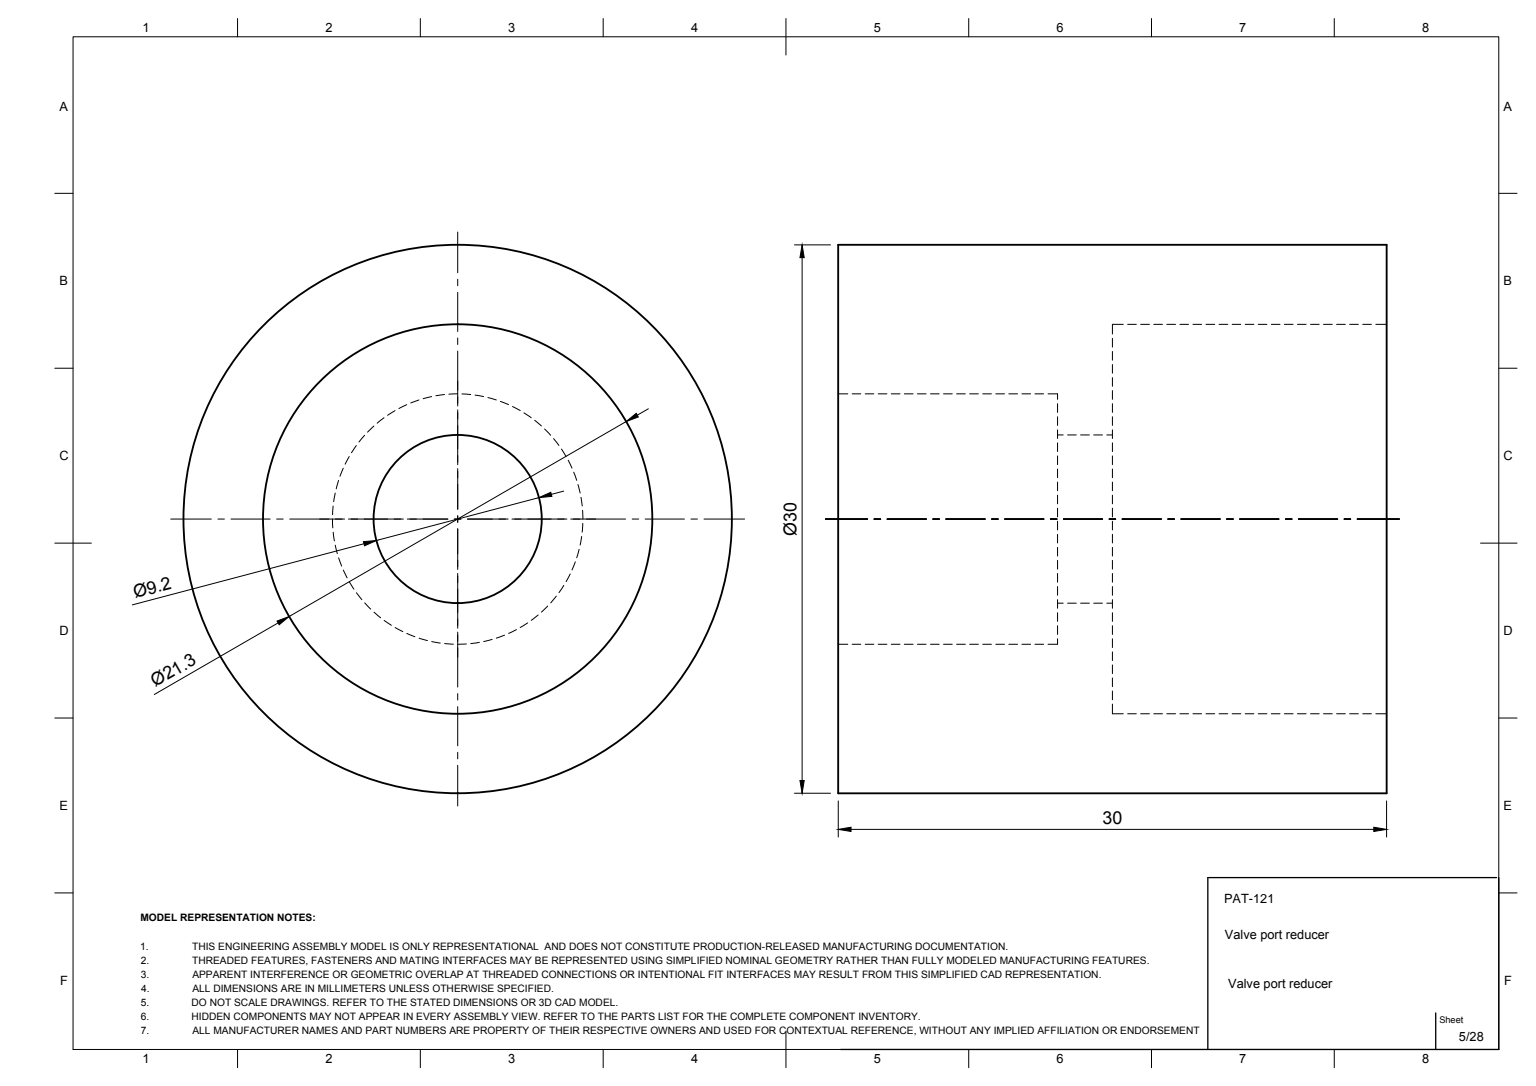
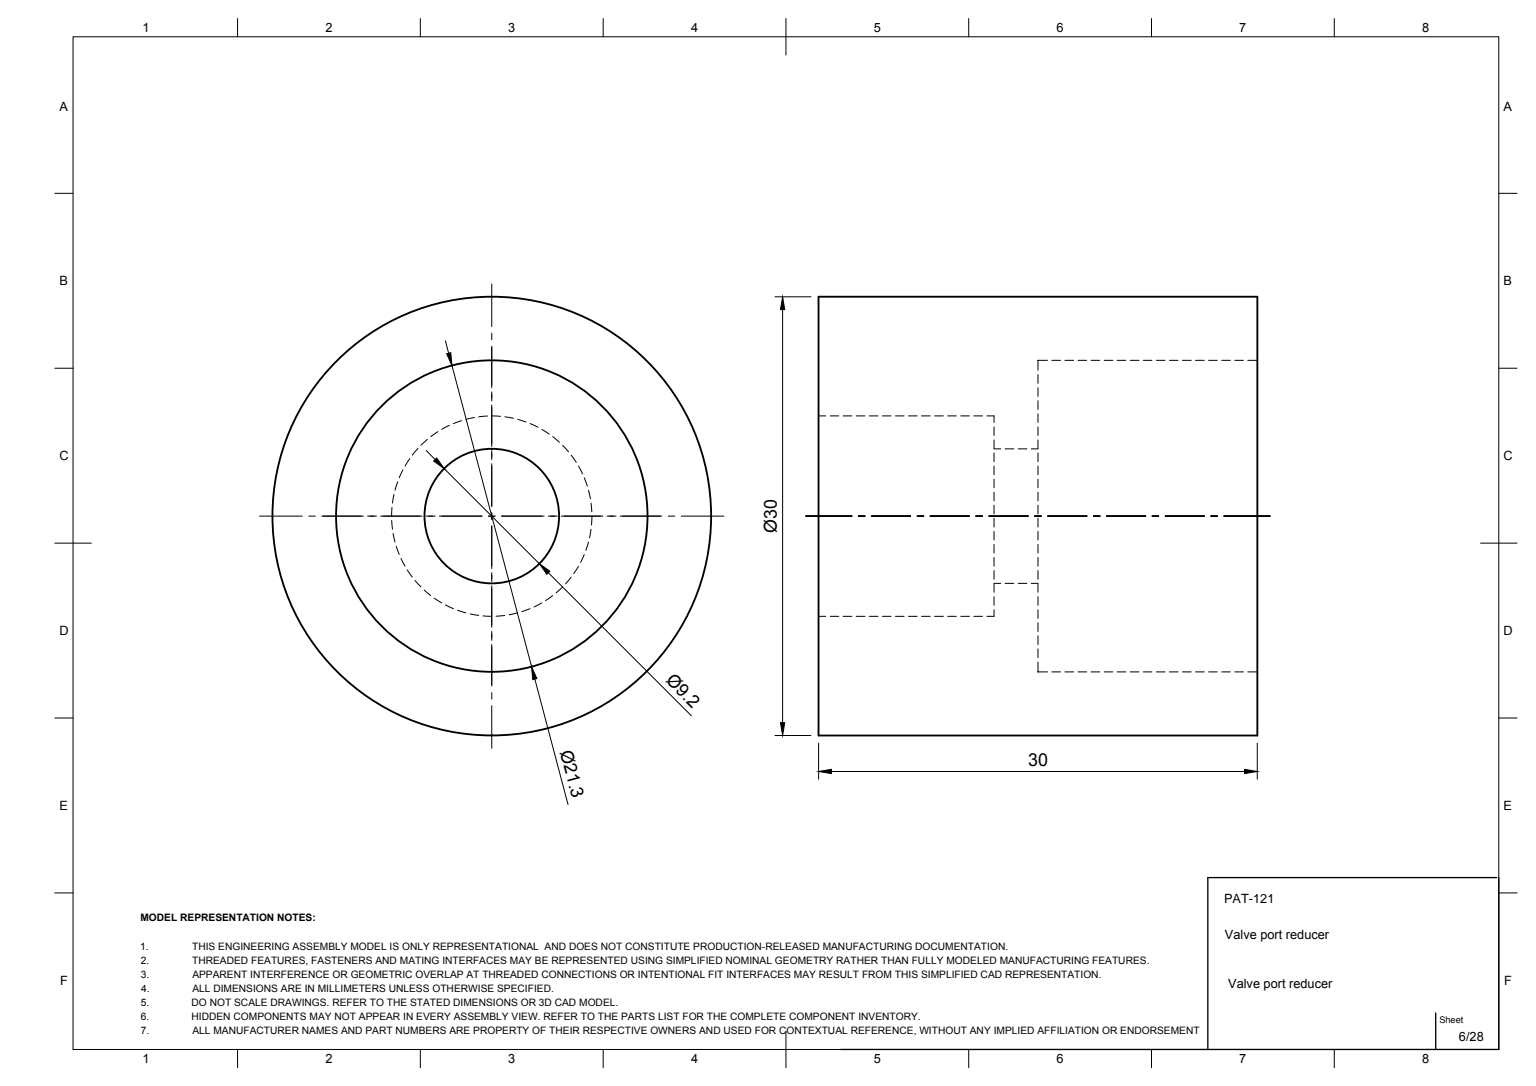
ISO-10303-21;
HEADER;
/* Generated by software containing ST-Developer
 * from STEP Tools, Inc. (www.steptools.com) 
 */

FILE_DESCRIPTION(
/* description */ ('Wall-mounted air drop station'),
/* implementation_level */ '2;1');

FILE_NAME(
/* name */ 'Valve port reducer.step',
/* time_stamp */ '2026-10-28T22:16:19-07:00',
/* author */ (''),
/* organization */ (''),
/* preprocessor_version */ 'ST-DEVELOPER v20.2',
/* originating_system */ 'Autodesk Translation Framework v15.17.0.0',
/* authorisation */ '');

FILE_SCHEMA (('AUTOMOTIVE_DESIGN { 1 0 10303 214 3 1 1 }'));
ENDSEC;

DATA;
#10=MECHANICAL_DESIGN_GEOMETRIC_PRESENTATION_REPRESENTATION('',(#344),#10517);
#286=SHAPE_REPRESENTATION_RELATIONSHIP('SRR','None',#10643,#315);
#315=ADVANCED_BREP_SHAPE_REPRESENTATION('',(#373),#10487);
#344=STYLED_ITEM('',(#10860),#373);
#373=MANIFOLD_SOLID_BREP('Body1',#5883);
#399=FACE_BOUND('',#1112,.T.);
#400=FACE_BOUND('',#1115,.T.);
#401=FACE_BOUND('',#1119,.T.);
#402=FACE_BOUND('',#1121,.T.);
#526=PLANE('',#6241);
#527=PLANE('',#6246);
#528=PLANE('',#6252);
#529=PLANE('',#6253);
#755=FACE_OUTER_BOUND('',#1110,.T.);
#756=FACE_OUTER_BOUND('',#1111,.T.);
#757=FACE_OUTER_BOUND('',#1113,.T.);
#758=FACE_OUTER_BOUND('',#1114,.T.);
#759=FACE_OUTER_BOUND('',#1116,.T.);
#760=FACE_OUTER_BOUND('',#1117,.T.);
#761=FACE_OUTER_BOUND('',#1118,.T.);
#762=FACE_OUTER_BOUND('',#1120,.T.);
#1110=EDGE_LOOP('',(#3973,#3974,#3975,#3976));
#1111=EDGE_LOOP('',(#3977));
#1112=EDGE_LOOP('',(#3978));
#1113=EDGE_LOOP('',(#3979,#3980,#3981,#3982));
#1114=EDGE_LOOP('',(#3983));
#1115=EDGE_LOOP('',(#3984));
#1116=EDGE_LOOP('',(#3985,#3986,#3987,#3988));
#1117=EDGE_LOOP('',(#3989,#3990,#3991,#3992));
#1118=EDGE_LOOP('',(#3993));
#1119=EDGE_LOOP('',(#3994));
#1120=EDGE_LOOP('',(#3995));
#1121=EDGE_LOOP('',(#3996));
#1592=LINE('',#8773,#2056);
#1593=LINE('',#8782,#2057);
#1594=LINE('',#8788,#2058);
#1595=LINE('',#8793,#2059);
#2056=VECTOR('',#6934,0.685);
#2057=VECTOR('',#6945,1.065);
#2058=VECTOR('',#6954,0.46);
#2059=VECTOR('',#6959,1.5);
#2520=CIRCLE('',#6239,0.685);
#2521=CIRCLE('',#6240,0.685);
#2522=CIRCLE('',#6242,0.46);
#2523=CIRCLE('',#6244,1.065);
#2524=CIRCLE('',#6245,1.065);
#2525=CIRCLE('',#6247,0.46);
#2526=CIRCLE('',#6250,1.5);
#2527=CIRCLE('',#6251,1.5);
#2765=VERTEX_POINT('',#8770);
#2766=VERTEX_POINT('',#8772);
#2767=VERTEX_POINT('',#8776);
#2768=VERTEX_POINT('',#8779);
#2769=VERTEX_POINT('',#8781);
#2770=VERTEX_POINT('',#8785);
#2771=VERTEX_POINT('',#8790);
#2772=VERTEX_POINT('',#8792);
#3244=EDGE_CURVE('',#2765,#2765,#2520,.T.);
#3245=EDGE_CURVE('',#2765,#2766,#1592,.T.);
#3246=EDGE_CURVE('',#2766,#2766,#2521,.T.);
#3247=EDGE_CURVE('',#2767,#2767,#2522,.T.);
#3248=EDGE_CURVE('',#2768,#2768,#2523,.T.);
#3249=EDGE_CURVE('',#2768,#2769,#1593,.T.);
#3250=EDGE_CURVE('',#2769,#2769,#2524,.T.);
#3251=EDGE_CURVE('',#2770,#2770,#2525,.T.);
#3252=EDGE_CURVE('',#2770,#2767,#1594,.T.);
#3253=EDGE_CURVE('',#2771,#2771,#2526,.T.);
#3254=EDGE_CURVE('',#2771,#2772,#1595,.T.);
#3255=EDGE_CURVE('',#2772,#2772,#2527,.T.);
#3973=ORIENTED_EDGE('',*,*,#3244,.F.);
#3974=ORIENTED_EDGE('',*,*,#3245,.T.);
#3975=ORIENTED_EDGE('',*,*,#3246,.T.);
#3976=ORIENTED_EDGE('',*,*,#3245,.F.);
#3977=ORIENTED_EDGE('',*,*,#3246,.F.);
#3978=ORIENTED_EDGE('',*,*,#3247,.F.);
#3979=ORIENTED_EDGE('',*,*,#3248,.F.);
#3980=ORIENTED_EDGE('',*,*,#3249,.T.);
#3981=ORIENTED_EDGE('',*,*,#3250,.F.);
#3982=ORIENTED_EDGE('',*,*,#3249,.F.);
#3983=ORIENTED_EDGE('',*,*,#3248,.T.);
#3984=ORIENTED_EDGE('',*,*,#3251,.F.);
#3985=ORIENTED_EDGE('',*,*,#3251,.T.);
#3986=ORIENTED_EDGE('',*,*,#3252,.T.);
#3987=ORIENTED_EDGE('',*,*,#3247,.T.);
#3988=ORIENTED_EDGE('',*,*,#3252,.F.);
#3989=ORIENTED_EDGE('',*,*,#3253,.F.);
#3990=ORIENTED_EDGE('',*,*,#3254,.T.);
#3991=ORIENTED_EDGE('',*,*,#3255,.T.);
#3992=ORIENTED_EDGE('',*,*,#3254,.F.);
#3993=ORIENTED_EDGE('',*,*,#3253,.T.);
#3994=ORIENTED_EDGE('',*,*,#3250,.T.);
#3995=ORIENTED_EDGE('',*,*,#3255,.F.);
#3996=ORIENTED_EDGE('',*,*,#3244,.T.);
#5431=CYLINDRICAL_SURFACE('',#6238,0.685);
#5432=CYLINDRICAL_SURFACE('',#6243,1.065);
#5433=CYLINDRICAL_SURFACE('',#6248,0.46);
#5434=CYLINDRICAL_SURFACE('',#6249,1.5);
#5528=ADVANCED_FACE('',(#755),#5431,.F.);
#5529=ADVANCED_FACE('',(#756,#399),#526,.F.);
#5530=ADVANCED_FACE('',(#757),#5432,.F.);
#5531=ADVANCED_FACE('',(#758,#400),#527,.T.);
#5532=ADVANCED_FACE('',(#759),#5433,.F.);
#5533=ADVANCED_FACE('',(#760),#5434,.T.);
#5534=ADVANCED_FACE('',(#761,#401),#528,.T.);
#5535=ADVANCED_FACE('',(#762,#402),#529,.F.);
#5883=CLOSED_SHELL('',(#5528,#5529,#5530,#5531,#5532,#5533,#5534,#5535));
#6237=AXIS2_PLACEMENT_3D('',#8768,#6928,#6929);
#6238=AXIS2_PLACEMENT_3D('',#8769,#6930,#6931);
#6239=AXIS2_PLACEMENT_3D('',#8771,#6932,#6933);
#6240=AXIS2_PLACEMENT_3D('',#8774,#6935,#6936);
#6241=AXIS2_PLACEMENT_3D('',#8775,#6937,#6938);
#6242=AXIS2_PLACEMENT_3D('',#8777,#6939,#6940);
#6243=AXIS2_PLACEMENT_3D('',#8778,#6941,#6942);
#6244=AXIS2_PLACEMENT_3D('',#8780,#6943,#6944);
#6245=AXIS2_PLACEMENT_3D('',#8783,#6946,#6947);
#6246=AXIS2_PLACEMENT_3D('',#8784,#6948,#6949);
#6247=AXIS2_PLACEMENT_3D('',#8786,#6950,#6951);
#6248=AXIS2_PLACEMENT_3D('',#8787,#6952,#6953);
#6249=AXIS2_PLACEMENT_3D('',#8789,#6955,#6956);
#6250=AXIS2_PLACEMENT_3D('',#8791,#6957,#6958);
#6251=AXIS2_PLACEMENT_3D('',#8794,#6960,#6961);
#6252=AXIS2_PLACEMENT_3D('',#8795,#6962,#6963);
#6253=AXIS2_PLACEMENT_3D('',#8796,#6964,#6965);
#6928=DIRECTION('axis',(0.,0.,1.));
#6929=DIRECTION('refdir',(1.,0.,0.));
#6930=DIRECTION('center_axis',(0.,1.,0.));
#6931=DIRECTION('ref_axis',(1.,0.,0.));
#6932=DIRECTION('center_axis',(0.,1.,0.));
#6933=DIRECTION('ref_axis',(1.,0.,0.));
#6934=DIRECTION('',(0.,1.,0.));
#6935=DIRECTION('center_axis',(0.,1.,0.));
#6936=DIRECTION('ref_axis',(1.,0.,0.));
#6937=DIRECTION('center_axis',(0.,1.,0.));
#6938=DIRECTION('ref_axis',(1.,0.,0.));
#6939=DIRECTION('center_axis',(0.,-1.,0.));
#6940=DIRECTION('ref_axis',(1.,0.,0.));
#6941=DIRECTION('center_axis',(0.,1.,0.));
#6942=DIRECTION('ref_axis',(1.,0.,0.));
#6943=DIRECTION('center_axis',(0.,1.,0.));
#6944=DIRECTION('ref_axis',(1.,0.,0.));
#6945=DIRECTION('',(0.,1.,0.));
#6946=DIRECTION('center_axis',(0.,-1.,0.));
#6947=DIRECTION('ref_axis',(1.,0.,0.));
#6948=DIRECTION('center_axis',(0.,1.,0.));
#6949=DIRECTION('ref_axis',(1.,0.,0.));
#6950=DIRECTION('center_axis',(0.,1.,0.));
#6951=DIRECTION('ref_axis',(1.,0.,0.));
#6952=DIRECTION('center_axis',(0.,1.,0.));
#6953=DIRECTION('ref_axis',(1.,0.,0.));
#6954=DIRECTION('',(0.,-1.,0.));
#6955=DIRECTION('center_axis',(0.,1.,0.));
#6956=DIRECTION('ref_axis',(1.,0.,0.));
#6957=DIRECTION('center_axis',(0.,1.,0.));
#6958=DIRECTION('ref_axis',(1.,0.,0.));
#6959=DIRECTION('',(0.,-1.,0.));
#6960=DIRECTION('center_axis',(0.,1.,0.));
#6961=DIRECTION('ref_axis',(1.,0.,0.));
#6962=DIRECTION('center_axis',(0.,1.,0.));
#6963=DIRECTION('ref_axis',(1.,0.,0.));
#6964=DIRECTION('center_axis',(0.,1.,0.));
#6965=DIRECTION('ref_axis',(1.,0.,0.));
#8768=CARTESIAN_POINT('',(0.,0.,0.));
#8769=CARTESIAN_POINT('Origin',(0.,-8.6,5.));
#8770=CARTESIAN_POINT('',(-0.685,-8.5,5.));
#8771=CARTESIAN_POINT('Origin',(0.,-8.5,5.));
#8772=CARTESIAN_POINT('',(-0.685,-7.3,5.));
#8773=CARTESIAN_POINT('',(-0.685,-8.6,5.));
#8774=CARTESIAN_POINT('Origin',(0.,-7.3,5.));
#8775=CARTESIAN_POINT('Origin',(0.,-7.3,5.));
#8776=CARTESIAN_POINT('',(-0.46,-7.3,5.));
#8777=CARTESIAN_POINT('Origin',(0.,-7.3,5.));
#8778=CARTESIAN_POINT('Origin',(0.,-7.,5.));
#8779=CARTESIAN_POINT('',(-1.065,-7.,5.));
#8780=CARTESIAN_POINT('Origin',(0.,-7.,5.));
#8781=CARTESIAN_POINT('',(-1.065,-5.5,5.));
#8782=CARTESIAN_POINT('',(-1.065,-7.,5.));
#8783=CARTESIAN_POINT('Origin',(0.,-5.5,5.));
#8784=CARTESIAN_POINT('Origin',(0.,-7.,5.));
#8785=CARTESIAN_POINT('',(-0.46,-7.,5.));
#8786=CARTESIAN_POINT('Origin',(0.,-7.,5.));
#8787=CARTESIAN_POINT('Origin',(0.,-8.5,5.));
#8788=CARTESIAN_POINT('',(-0.46,-8.5,5.));
#8789=CARTESIAN_POINT('Origin',(0.,-8.5,5.));
#8790=CARTESIAN_POINT('',(-1.5,-5.5,5.));
#8791=CARTESIAN_POINT('Origin',(0.,-5.5,5.));
#8792=CARTESIAN_POINT('',(-1.5,-8.5,5.));
#8793=CARTESIAN_POINT('',(-1.5,-8.5,5.));
#8794=CARTESIAN_POINT('Origin',(0.,-8.5,5.));
#8795=CARTESIAN_POINT('Origin',(0.,-5.5,5.));
#8796=CARTESIAN_POINT('Origin',(0.,-8.5,5.));
#10454=UNCERTAINTY_MEASURE_WITH_UNIT(LENGTH_MEASURE(0.001),#10518,
'DISTANCE_ACCURACY_VALUE',
'Maximum model space distance between geometric entities at asserted c
onnectivities');
#10484=UNCERTAINTY_MEASURE_WITH_UNIT(LENGTH_MEASURE(0.001),#10518,
'DISTANCE_ACCURACY_VALUE',
'Maximum model space distance between geometric entities at asserted c
onnectivities');
#10487=(
GEOMETRIC_REPRESENTATION_CONTEXT(3)
GLOBAL_UNCERTAINTY_ASSIGNED_CONTEXT((#10454))
GLOBAL_UNIT_ASSIGNED_CONTEXT((#10518,#10520,#10521))
REPRESENTATION_CONTEXT('','3D')
);
#10517=(
GEOMETRIC_REPRESENTATION_CONTEXT(3)
GLOBAL_UNCERTAINTY_ASSIGNED_CONTEXT((#10484))
GLOBAL_UNIT_ASSIGNED_CONTEXT((#10518,#10520,#10521))
REPRESENTATION_CONTEXT('','3D')
);
#10518=(
LENGTH_UNIT()
NAMED_UNIT(*)
SI_UNIT(.CENTI.,.METRE.)
);
#10520=(
NAMED_UNIT(*)
PLANE_ANGLE_UNIT()
SI_UNIT($,.RADIAN.)
);
#10521=(
NAMED_UNIT(*)
SI_UNIT($,.STERADIAN.)
SOLID_ANGLE_UNIT()
);
#10524=SHAPE_DEFINITION_REPRESENTATION(#10556,#10643);
#10556=PRODUCT_DEFINITION_SHAPE('',$,#10676);
#10643=SHAPE_REPRESENTATION('',(#6237),#10487);
#10673=PRODUCT_DEFINITION_CONTEXT('part definition',#10771,'design');
#10676=PRODUCT_DEFINITION('Valve port reducer','Valve port reducer',#10708,
#10673);
#10708=PRODUCT_DEFINITION_FORMATION('',$,#10775);
#10771=APPLICATION_CONTEXT(
'Core Data for Automotive Mechanical Design Process');
#10772=PRODUCT_CONTEXT('part definition',#10771,'mechanical');
#10775=PRODUCT('Valve port reducer','Valve port reducer',
'Valve port reducer',(#10772));
#10854=COLOUR_RGB('Light Blue',0.38,0.62,0.78);
#10855=FILL_AREA_STYLE_COLOUR('',#10854);
#10856=FILL_AREA_STYLE('',(#10855));
#10857=SURFACE_STYLE_FILL_AREA(#10856);
#10858=SURFACE_SIDE_STYLE('',(#10857));
#10859=SURFACE_STYLE_USAGE(.BOTH.,#10858);
#10860=PRESENTATION_STYLE_ASSIGNMENT((#10859));
ENDSEC;
END-ISO-10303-21;
